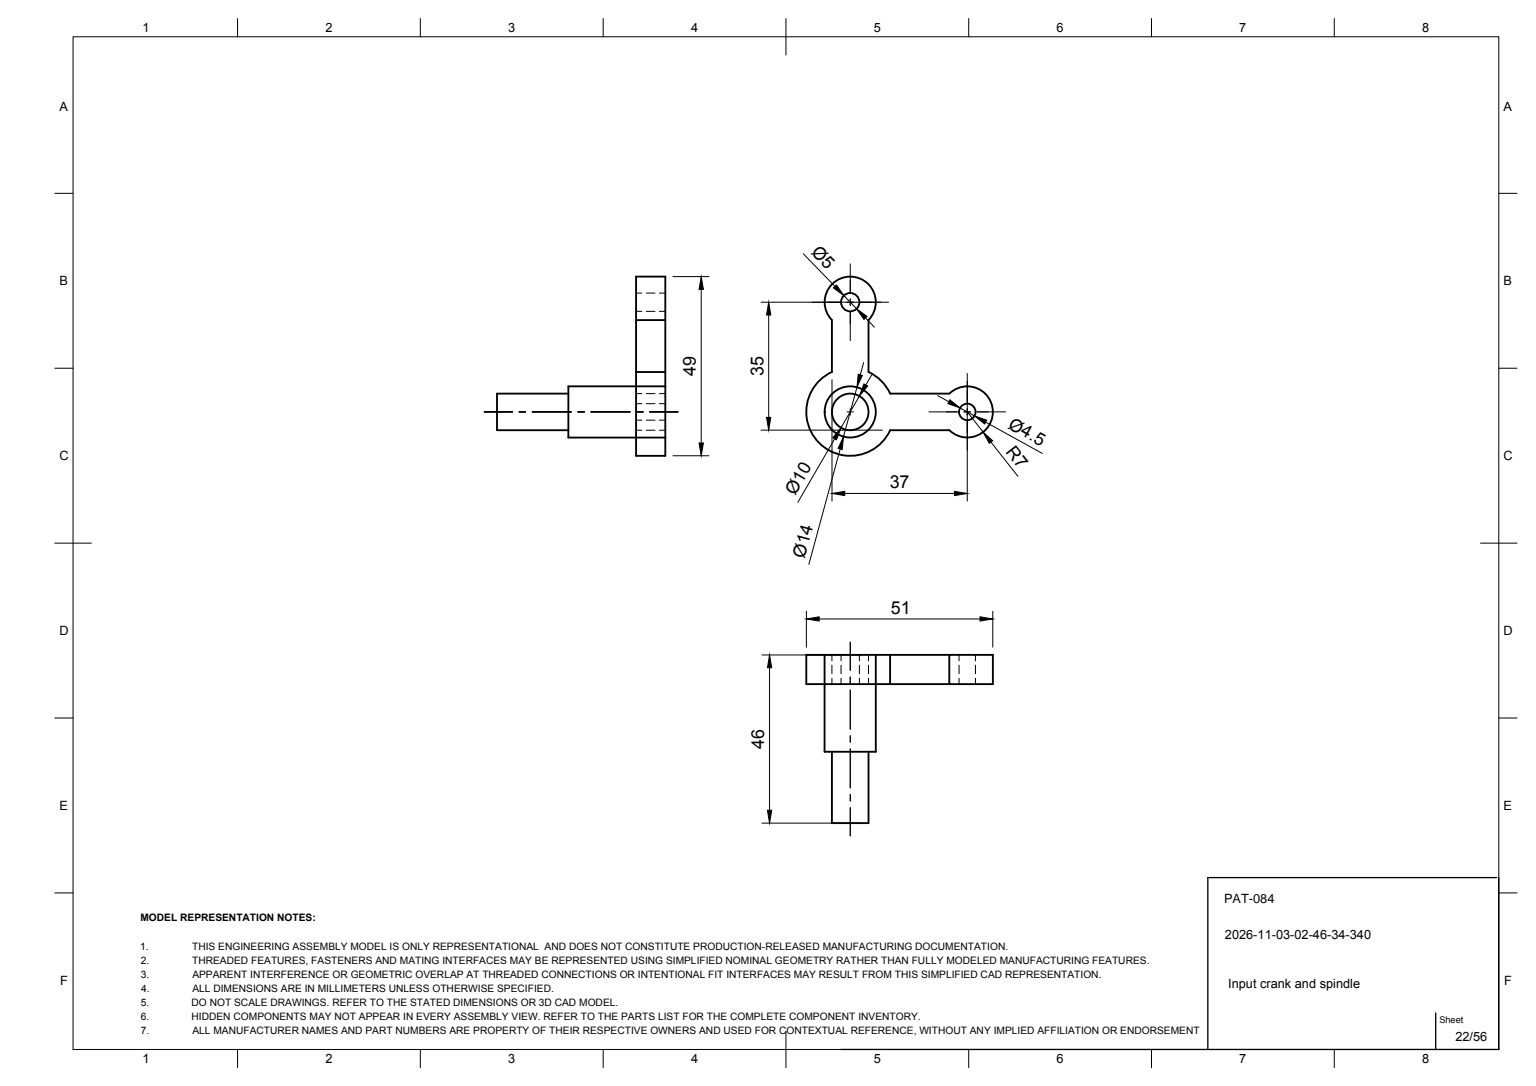
ISO-10303-21;
HEADER;
/* Generated by software containing ST-Developer
 * from STEP Tools, Inc. (www.steptools.com) 
 */

FILE_DESCRIPTION(
/* description */ ('Quick-return (Whitworth) mechanism'),
/* implementation_level */ '2;1');

FILE_NAME(
/* name */ 'Input crank and spindle.step',
/* time_stamp */ '2026-10-28T03:25:57-07:00',
/* author */ (''),
/* organization */ (''),
/* preprocessor_version */ 'ST-DEVELOPER v20.2',
/* originating_system */ 'Autodesk Translation Framework v15.17.0.0',
/* authorisation */ '');

FILE_SCHEMA (('AUTOMOTIVE_DESIGN { 1 0 10303 214 3 1 1 }'));
ENDSEC;

DATA;
#10=MECHANICAL_DESIGN_GEOMETRIC_PRESENTATION_REPRESENTATION('',(#511),#14878);
#415=SHAPE_REPRESENTATION_RELATIONSHIP('SRR','None',#15085,#459);
#459=ADVANCED_BREP_SHAPE_REPRESENTATION('',(#563),#14842);
#511=STYLED_ITEM('',(#15399),#563);
#563=MANIFOLD_SOLID_BREP('Body1',#7865);
#702=FACE_BOUND('',#1829,.T.);
#703=FACE_BOUND('',#1830,.T.);
#704=FACE_BOUND('',#1831,.T.);
#705=FACE_BOUND('',#1838,.T.);
#706=FACE_BOUND('',#1839,.T.);
#707=FACE_BOUND('',#1843,.T.);
#873=PLANE('',#8850);
#874=PLANE('',#8851);
#875=PLANE('',#8857);
#876=PLANE('',#8864);
#877=PLANE('',#8865);
#878=PLANE('',#8867);
#879=PLANE('',#8869);
#880=PLANE('',#8875);
#1248=FACE_OUTER_BOUND('',#1825,.T.);
#1249=FACE_OUTER_BOUND('',#1826,.T.);
#1250=FACE_OUTER_BOUND('',#1827,.T.);
#1251=FACE_OUTER_BOUND('',#1828,.T.);
#1252=FACE_OUTER_BOUND('',#1832,.T.);
#1253=FACE_OUTER_BOUND('',#1833,.T.);
#1254=FACE_OUTER_BOUND('',#1834,.T.);
#1255=FACE_OUTER_BOUND('',#1835,.T.);
#1256=FACE_OUTER_BOUND('',#1836,.T.);
#1257=FACE_OUTER_BOUND('',#1837,.T.);
#1258=FACE_OUTER_BOUND('',#1840,.T.);
#1259=FACE_OUTER_BOUND('',#1841,.T.);
#1260=FACE_OUTER_BOUND('',#1842,.T.);
#1261=FACE_OUTER_BOUND('',#1844,.T.);
#1262=FACE_OUTER_BOUND('',#1845,.T.);
#1263=FACE_OUTER_BOUND('',#1846,.T.);
#1825=EDGE_LOOP('',(#6130,#6131,#6132,#6133));
#1826=EDGE_LOOP('',(#6134,#6135,#6136,#6137));
#1827=EDGE_LOOP('',(#6138,#6139,#6140,#6141));
#1828=EDGE_LOOP('',(#6142,#6143,#6144,#6145,#6146,#6147,#6148,#6149));
#1829=EDGE_LOOP('',(#6150));
#1830=EDGE_LOOP('',(#6151));
#1831=EDGE_LOOP('',(#6152));
#1832=EDGE_LOOP('',(#6153,#6154,#6155,#6156));
#1833=EDGE_LOOP('',(#6157,#6158,#6159,#6160));
#1834=EDGE_LOOP('',(#6161,#6162,#6163,#6164));
#1835=EDGE_LOOP('',(#6165,#6166,#6167,#6168));
#1836=EDGE_LOOP('',(#6169,#6170,#6171,#6172));
#1837=EDGE_LOOP('',(#6173,#6174,#6175,#6176,#6177,#6178,#6179,#6180));
#1838=EDGE_LOOP('',(#6181));
#1839=EDGE_LOOP('',(#6182));
#1840=EDGE_LOOP('',(#6183,#6184,#6185,#6186));
#1841=EDGE_LOOP('',(#6187,#6188,#6189,#6190));
#1842=EDGE_LOOP('',(#6191));
#1843=EDGE_LOOP('',(#6192));
#1844=EDGE_LOOP('',(#6193,#6194,#6195,#6196));
#1845=EDGE_LOOP('',(#6197,#6198,#6199,#6200));
#1846=EDGE_LOOP('',(#6201));
#2342=LINE('',#13382,#2865);
#2343=LINE('',#13387,#2866);
#2344=LINE('',#13391,#2867);
#2345=LINE('',#13395,#2868);
#2346=LINE('',#13397,#2869);
#2347=LINE('',#13398,#2870);
#2348=LINE('',#13401,#2871);
#2349=LINE('',#13405,#2872);
#2350=LINE('',#13409,#2873);
#2351=LINE('',#13417,#2874);
#2352=LINE('',#13418,#2875);
#2353=LINE('',#13422,#2876);
#2354=LINE('',#13425,#2877);
#2355=LINE('',#13429,#2878);
#2356=LINE('',#13431,#2879);
#2357=LINE('',#13435,#2880);
#2358=LINE('',#13436,#2881);
#2359=LINE('',#13439,#2882);
#2360=LINE('',#13448,#2883);
#2361=LINE('',#13451,#2884);
#2865=VECTOR('',#10493,0.225);
#2866=VECTOR('',#10498,1.);
#2867=VECTOR('',#10501,1.);
#2868=VECTOR('',#10506,1.);
#2869=VECTOR('',#10507,1.);
#2870=VECTOR('',#10508,1.);
#2871=VECTOR('',#10511,1.);
#2872=VECTOR('',#10514,1.);
#2873=VECTOR('',#10517,1.);
#2874=VECTOR('',#10526,1.);
#2875=VECTOR('',#10527,1.);
#2876=VECTOR('',#10532,1.);
#2877=VECTOR('',#10535,0.25);
#2878=VECTOR('',#10540,1.);
#2879=VECTOR('',#10541,1.);
#2880=VECTOR('',#10546,1.);
#2881=VECTOR('',#10547,1.);
#2882=VECTOR('',#10552,1.);
#2883=VECTOR('',#10565,0.7);
#2884=VECTOR('',#10568,0.5);
#3452=CIRCLE('',#8845,0.225);
#3453=CIRCLE('',#8846,0.225);
#3454=CIRCLE('',#8848,0.7);
#3455=CIRCLE('',#8849,0.7);
#3456=CIRCLE('',#8852,1.2);
#3457=CIRCLE('',#8853,0.7);
#3458=CIRCLE('',#8854,1.2);
#3459=CIRCLE('',#8855,0.25);
#3460=CIRCLE('',#8856,0.7);
#3461=CIRCLE('',#8859,1.2);
#3462=CIRCLE('',#8861,0.25);
#3463=CIRCLE('',#8863,0.7);
#3464=CIRCLE('',#8866,1.2);
#3465=CIRCLE('',#8870,0.7);
#3466=CIRCLE('',#8871,0.5);
#3467=CIRCLE('',#8874,0.5);
#3931=VERTEX_POINT('',#13379);
#3932=VERTEX_POINT('',#13381);
#3933=VERTEX_POINT('',#13385);
#3934=VERTEX_POINT('',#13386);
#3935=VERTEX_POINT('',#13388);
#3936=VERTEX_POINT('',#13390);
#3937=VERTEX_POINT('',#13394);
#3938=VERTEX_POINT('',#13396);
#3939=VERTEX_POINT('',#13400);
#3940=VERTEX_POINT('',#13402);
#3941=VERTEX_POINT('',#13404);
#3942=VERTEX_POINT('',#13406);
#3943=VERTEX_POINT('',#13408);
#3944=VERTEX_POINT('',#13411);
#3945=VERTEX_POINT('',#13413);
#3946=VERTEX_POINT('',#13416);
#3947=VERTEX_POINT('',#13420);
#3948=VERTEX_POINT('',#13424);
#3949=VERTEX_POINT('',#13428);
#3950=VERTEX_POINT('',#13430);
#3951=VERTEX_POINT('',#13434);
#3952=VERTEX_POINT('',#13443);
#3953=VERTEX_POINT('',#13445);
#3954=VERTEX_POINT('',#13450);
#4722=EDGE_CURVE('',#3931,#3931,#3452,.T.);
#4723=EDGE_CURVE('',#3931,#3932,#2342,.T.);
#4724=EDGE_CURVE('',#3932,#3932,#3453,.T.);
#4725=EDGE_CURVE('',#3933,#3934,#2343,.T.);
#4726=EDGE_CURVE('',#3935,#3933,#3454,.T.);
#4727=EDGE_CURVE('',#3936,#3935,#2344,.T.);
#4728=EDGE_CURVE('',#3936,#3934,#3455,.T.);
#4729=EDGE_CURVE('',#3937,#3934,#2345,.T.);
#4730=EDGE_CURVE('',#3938,#3937,#2346,.T.);
#4731=EDGE_CURVE('',#3933,#3938,#2347,.T.);
#4732=EDGE_CURVE('',#3936,#3939,#2348,.T.);
#4733=EDGE_CURVE('',#3940,#3939,#3456,.T.);
#4734=EDGE_CURVE('',#3940,#3941,#2349,.T.);
#4735=EDGE_CURVE('',#3942,#3941,#3457,.T.);
#4736=EDGE_CURVE('',#3942,#3943,#2350,.T.);
#4737=EDGE_CURVE('',#3937,#3943,#3458,.T.);
#4738=EDGE_CURVE('',#3944,#3944,#3459,.T.);
#4739=EDGE_CURVE('',#3945,#3945,#3460,.T.);
#4740=EDGE_CURVE('',#3946,#3935,#2351,.T.);
#4741=EDGE_CURVE('',#3939,#3946,#2352,.T.);
#4742=EDGE_CURVE('',#3947,#3946,#3461,.T.);
#4743=EDGE_CURVE('',#3947,#3940,#2353,.T.);
#4744=EDGE_CURVE('',#3944,#3948,#2354,.T.);
#4745=EDGE_CURVE('',#3948,#3948,#3462,.T.);
#4746=EDGE_CURVE('',#3942,#3949,#2355,.T.);
#4747=EDGE_CURVE('',#3950,#3941,#2356,.T.);
#4748=EDGE_CURVE('',#3949,#3950,#3463,.T.);
#4749=EDGE_CURVE('',#3951,#3949,#2357,.T.);
#4750=EDGE_CURVE('',#3943,#3951,#2358,.T.);
#4751=EDGE_CURVE('',#3938,#3951,#3464,.T.);
#4752=EDGE_CURVE('',#3950,#3947,#2359,.T.);
#4753=EDGE_CURVE('',#3952,#3952,#3465,.T.);
#4754=EDGE_CURVE('',#3953,#3953,#3466,.T.);
#4755=EDGE_CURVE('',#3945,#3952,#2360,.T.);
#4756=EDGE_CURVE('',#3953,#3954,#2361,.T.);
#4757=EDGE_CURVE('',#3954,#3954,#3467,.T.);
#6130=ORIENTED_EDGE('',*,*,#4722,.F.);
#6131=ORIENTED_EDGE('',*,*,#4723,.T.);
#6132=ORIENTED_EDGE('',*,*,#4724,.F.);
#6133=ORIENTED_EDGE('',*,*,#4723,.F.);
#6134=ORIENTED_EDGE('',*,*,#4725,.F.);
#6135=ORIENTED_EDGE('',*,*,#4726,.F.);
#6136=ORIENTED_EDGE('',*,*,#4727,.F.);
#6137=ORIENTED_EDGE('',*,*,#4728,.T.);
#6138=ORIENTED_EDGE('',*,*,#4725,.T.);
#6139=ORIENTED_EDGE('',*,*,#4729,.F.);
#6140=ORIENTED_EDGE('',*,*,#4730,.F.);
#6141=ORIENTED_EDGE('',*,*,#4731,.F.);
#6142=ORIENTED_EDGE('',*,*,#4728,.F.);
#6143=ORIENTED_EDGE('',*,*,#4732,.T.);
#6144=ORIENTED_EDGE('',*,*,#4733,.F.);
#6145=ORIENTED_EDGE('',*,*,#4734,.T.);
#6146=ORIENTED_EDGE('',*,*,#4735,.F.);
#6147=ORIENTED_EDGE('',*,*,#4736,.T.);
#6148=ORIENTED_EDGE('',*,*,#4737,.F.);
#6149=ORIENTED_EDGE('',*,*,#4729,.T.);
#6150=ORIENTED_EDGE('',*,*,#4722,.T.);
#6151=ORIENTED_EDGE('',*,*,#4738,.T.);
#6152=ORIENTED_EDGE('',*,*,#4739,.T.);
#6153=ORIENTED_EDGE('',*,*,#4727,.T.);
#6154=ORIENTED_EDGE('',*,*,#4740,.F.);
#6155=ORIENTED_EDGE('',*,*,#4741,.F.);
#6156=ORIENTED_EDGE('',*,*,#4732,.F.);
#6157=ORIENTED_EDGE('',*,*,#4741,.T.);
#6158=ORIENTED_EDGE('',*,*,#4742,.F.);
#6159=ORIENTED_EDGE('',*,*,#4743,.T.);
#6160=ORIENTED_EDGE('',*,*,#4733,.T.);
#6161=ORIENTED_EDGE('',*,*,#4738,.F.);
#6162=ORIENTED_EDGE('',*,*,#4744,.T.);
#6163=ORIENTED_EDGE('',*,*,#4745,.F.);
#6164=ORIENTED_EDGE('',*,*,#4744,.F.);
#6165=ORIENTED_EDGE('',*,*,#4746,.F.);
#6166=ORIENTED_EDGE('',*,*,#4735,.T.);
#6167=ORIENTED_EDGE('',*,*,#4747,.F.);
#6168=ORIENTED_EDGE('',*,*,#4748,.F.);
#6169=ORIENTED_EDGE('',*,*,#4746,.T.);
#6170=ORIENTED_EDGE('',*,*,#4749,.F.);
#6171=ORIENTED_EDGE('',*,*,#4750,.F.);
#6172=ORIENTED_EDGE('',*,*,#4736,.F.);
#6173=ORIENTED_EDGE('',*,*,#4731,.T.);
#6174=ORIENTED_EDGE('',*,*,#4751,.T.);
#6175=ORIENTED_EDGE('',*,*,#4749,.T.);
#6176=ORIENTED_EDGE('',*,*,#4748,.T.);
#6177=ORIENTED_EDGE('',*,*,#4752,.T.);
#6178=ORIENTED_EDGE('',*,*,#4742,.T.);
#6179=ORIENTED_EDGE('',*,*,#4740,.T.);
#6180=ORIENTED_EDGE('',*,*,#4726,.T.);
#6181=ORIENTED_EDGE('',*,*,#4724,.T.);
#6182=ORIENTED_EDGE('',*,*,#4745,.T.);
#6183=ORIENTED_EDGE('',*,*,#4747,.T.);
#6184=ORIENTED_EDGE('',*,*,#4734,.F.);
#6185=ORIENTED_EDGE('',*,*,#4743,.F.);
#6186=ORIENTED_EDGE('',*,*,#4752,.F.);
#6187=ORIENTED_EDGE('',*,*,#4730,.T.);
#6188=ORIENTED_EDGE('',*,*,#4737,.T.);
#6189=ORIENTED_EDGE('',*,*,#4750,.T.);
#6190=ORIENTED_EDGE('',*,*,#4751,.F.);
#6191=ORIENTED_EDGE('',*,*,#4753,.F.);
#6192=ORIENTED_EDGE('',*,*,#4754,.F.);
#6193=ORIENTED_EDGE('',*,*,#4739,.F.);
#6194=ORIENTED_EDGE('',*,*,#4755,.T.);
#6195=ORIENTED_EDGE('',*,*,#4753,.T.);
#6196=ORIENTED_EDGE('',*,*,#4755,.F.);
#6197=ORIENTED_EDGE('',*,*,#4754,.T.);
#6198=ORIENTED_EDGE('',*,*,#4756,.T.);
#6199=ORIENTED_EDGE('',*,*,#4757,.T.);
#6200=ORIENTED_EDGE('',*,*,#4756,.F.);
#6201=ORIENTED_EDGE('',*,*,#4757,.F.);
#7298=CYLINDRICAL_SURFACE('',#8844,0.225);
#7299=CYLINDRICAL_SURFACE('',#8847,0.7);
#7300=CYLINDRICAL_SURFACE('',#8858,1.2);
#7301=CYLINDRICAL_SURFACE('',#8860,0.25);
#7302=CYLINDRICAL_SURFACE('',#8862,0.7);
#7303=CYLINDRICAL_SURFACE('',#8868,1.2);
#7304=CYLINDRICAL_SURFACE('',#8872,0.7);
#7305=CYLINDRICAL_SURFACE('',#8873,0.5);
#7579=ADVANCED_FACE('',(#1248),#7298,.F.);
#7580=ADVANCED_FACE('',(#1249),#7299,.T.);
#7581=ADVANCED_FACE('',(#1250),#873,.T.);
#7582=ADVANCED_FACE('',(#1251,#702,#703,#704),#874,.F.);
#7583=ADVANCED_FACE('',(#1252),#875,.T.);
#7584=ADVANCED_FACE('',(#1253),#7300,.T.);
#7585=ADVANCED_FACE('',(#1254),#7301,.F.);
#7586=ADVANCED_FACE('',(#1255),#7302,.T.);
#7587=ADVANCED_FACE('',(#1256),#876,.T.);
#7588=ADVANCED_FACE('',(#1257,#705,#706),#877,.T.);
#7589=ADVANCED_FACE('',(#1258),#878,.T.);
#7590=ADVANCED_FACE('',(#1259),#7303,.T.);
#7591=ADVANCED_FACE('',(#1260,#707),#879,.F.);
#7592=ADVANCED_FACE('',(#1261),#7304,.T.);
#7593=ADVANCED_FACE('',(#1262),#7305,.T.);
#7594=ADVANCED_FACE('',(#1263),#880,.F.);
#7865=CLOSED_SHELL('',(#7579,#7580,#7581,#7582,#7583,#7584,#7585,#7586,
#7587,#7588,#7589,#7590,#7591,#7592,#7593,#7594));
#8843=AXIS2_PLACEMENT_3D('',#13377,#10487,#10488);
#8844=AXIS2_PLACEMENT_3D('',#13378,#10489,#10490);
#8845=AXIS2_PLACEMENT_3D('',#13380,#10491,#10492);
#8846=AXIS2_PLACEMENT_3D('',#13383,#10494,#10495);
#8847=AXIS2_PLACEMENT_3D('',#13384,#10496,#10497);
#8848=AXIS2_PLACEMENT_3D('',#13389,#10499,#10500);
#8849=AXIS2_PLACEMENT_3D('',#13392,#10502,#10503);
#8850=AXIS2_PLACEMENT_3D('',#13393,#10504,#10505);
#8851=AXIS2_PLACEMENT_3D('',#13399,#10509,#10510);
#8852=AXIS2_PLACEMENT_3D('',#13403,#10512,#10513);
#8853=AXIS2_PLACEMENT_3D('',#13407,#10515,#10516);
#8854=AXIS2_PLACEMENT_3D('',#13410,#10518,#10519);
#8855=AXIS2_PLACEMENT_3D('',#13412,#10520,#10521);
#8856=AXIS2_PLACEMENT_3D('',#13414,#10522,#10523);
#8857=AXIS2_PLACEMENT_3D('',#13415,#10524,#10525);
#8858=AXIS2_PLACEMENT_3D('',#13419,#10528,#10529);
#8859=AXIS2_PLACEMENT_3D('',#13421,#10530,#10531);
#8860=AXIS2_PLACEMENT_3D('',#13423,#10533,#10534);
#8861=AXIS2_PLACEMENT_3D('',#13426,#10536,#10537);
#8862=AXIS2_PLACEMENT_3D('',#13427,#10538,#10539);
#8863=AXIS2_PLACEMENT_3D('',#13432,#10542,#10543);
#8864=AXIS2_PLACEMENT_3D('',#13433,#10544,#10545);
#8865=AXIS2_PLACEMENT_3D('',#13437,#10548,#10549);
#8866=AXIS2_PLACEMENT_3D('',#13438,#10550,#10551);
#8867=AXIS2_PLACEMENT_3D('',#13440,#10553,#10554);
#8868=AXIS2_PLACEMENT_3D('',#13441,#10555,#10556);
#8869=AXIS2_PLACEMENT_3D('',#13442,#10557,#10558);
#8870=AXIS2_PLACEMENT_3D('',#13444,#10559,#10560);
#8871=AXIS2_PLACEMENT_3D('',#13446,#10561,#10562);
#8872=AXIS2_PLACEMENT_3D('',#13447,#10563,#10564);
#8873=AXIS2_PLACEMENT_3D('',#13449,#10566,#10567);
#8874=AXIS2_PLACEMENT_3D('',#13452,#10569,#10570);
#8875=AXIS2_PLACEMENT_3D('',#13453,#10571,#10572);
#10487=DIRECTION('axis',(0.,0.,1.));
#10488=DIRECTION('refdir',(1.,0.,0.));
#10489=DIRECTION('center_axis',(0.,0.,1.));
#10490=DIRECTION('ref_axis',(1.,0.,0.));
#10491=DIRECTION('center_axis',(0.,0.,1.));
#10492=DIRECTION('ref_axis',(1.,0.,0.));
#10493=DIRECTION('',(0.,0.,1.));
#10494=DIRECTION('center_axis',(0.,0.,-1.));
#10495=DIRECTION('ref_axis',(1.,0.,0.));
#10496=DIRECTION('center_axis',(0.,0.,1.));
#10497=DIRECTION('ref_axis',(-1.,-1.22464679914735E-16,0.));
#10498=DIRECTION('',(0.,0.,-1.));
#10499=DIRECTION('center_axis',(0.,0.,1.));
#10500=DIRECTION('ref_axis',(1.,0.,0.));
#10501=DIRECTION('',(0.,0.,1.));
#10502=DIRECTION('center_axis',(0.,0.,1.));
#10503=DIRECTION('ref_axis',(1.,0.,0.));
#10504=DIRECTION('center_axis',(0.,-1.,0.));
#10505=DIRECTION('ref_axis',(1.,0.,0.));
#10506=DIRECTION('',(-1.,0.,0.));
#10507=DIRECTION('',(0.,0.,-1.));
#10508=DIRECTION('',(1.,0.,0.));
#10509=DIRECTION('center_axis',(0.,0.,1.));
#10510=DIRECTION('ref_axis',(1.,0.,0.));
#10511=DIRECTION('',(1.,0.,0.));
#10512=DIRECTION('center_axis',(0.,0.,1.));
#10513=DIRECTION('ref_axis',(1.,0.,0.));
#10514=DIRECTION('',(0.,1.,0.));
#10515=DIRECTION('center_axis',(0.,0.,1.));
#10516=DIRECTION('ref_axis',(1.,0.,0.));
#10517=DIRECTION('',(0.,-1.,0.));
#10518=DIRECTION('center_axis',(0.,0.,1.));
#10519=DIRECTION('ref_axis',(1.,0.,0.));
#10520=DIRECTION('center_axis',(0.,0.,1.));
#10521=DIRECTION('ref_axis',(1.,0.,0.));
#10522=DIRECTION('center_axis',(0.,0.,1.));
#10523=DIRECTION('ref_axis',(1.,0.,0.));
#10524=DIRECTION('center_axis',(0.,1.,0.));
#10525=DIRECTION('ref_axis',(-1.,0.,0.));
#10526=DIRECTION('',(-1.,0.,0.));
#10527=DIRECTION('',(0.,0.,1.));
#10528=DIRECTION('center_axis',(0.,0.,1.));
#10529=DIRECTION('ref_axis',(1.,0.,0.));
#10530=DIRECTION('center_axis',(0.,0.,1.));
#10531=DIRECTION('ref_axis',(1.,0.,0.));
#10532=DIRECTION('',(0.,0.,-1.));
#10533=DIRECTION('center_axis',(0.,0.,1.));
#10534=DIRECTION('ref_axis',(1.,0.,0.));
#10535=DIRECTION('',(0.,0.,1.));
#10536=DIRECTION('center_axis',(0.,0.,-1.));
#10537=DIRECTION('ref_axis',(1.,0.,0.));
#10538=DIRECTION('center_axis',(0.,0.,1.));
#10539=DIRECTION('ref_axis',(6.12323399573677E-17,1.,0.));
#10540=DIRECTION('',(0.,0.,1.));
#10541=DIRECTION('',(0.,0.,-1.));
#10542=DIRECTION('center_axis',(0.,0.,1.));
#10543=DIRECTION('ref_axis',(1.,0.,0.));
#10544=DIRECTION('center_axis',(1.,0.,0.));
#10545=DIRECTION('ref_axis',(0.,1.,0.));
#10546=DIRECTION('',(0.,1.,0.));
#10547=DIRECTION('',(0.,0.,1.));
#10548=DIRECTION('center_axis',(0.,0.,1.));
#10549=DIRECTION('ref_axis',(1.,0.,0.));
#10550=DIRECTION('center_axis',(0.,0.,1.));
#10551=DIRECTION('ref_axis',(1.,0.,0.));
#10552=DIRECTION('',(0.,-1.,0.));
#10553=DIRECTION('center_axis',(-1.,0.,0.));
#10554=DIRECTION('ref_axis',(0.,-1.,0.));
#10555=DIRECTION('center_axis',(0.,0.,1.));
#10556=DIRECTION('ref_axis',(1.,0.,0.));
#10557=DIRECTION('center_axis',(0.,0.,1.));
#10558=DIRECTION('ref_axis',(1.,0.,0.));
#10559=DIRECTION('center_axis',(0.,0.,1.));
#10560=DIRECTION('ref_axis',(1.,0.,0.));
#10561=DIRECTION('center_axis',(0.,0.,-1.));
#10562=DIRECTION('ref_axis',(1.,0.,0.));
#10563=DIRECTION('center_axis',(0.,0.,1.));
#10564=DIRECTION('ref_axis',(1.,0.,0.));
#10565=DIRECTION('',(0.,0.,-1.));
#10566=DIRECTION('center_axis',(0.,0.,1.));
#10567=DIRECTION('ref_axis',(1.,0.,0.));
#10568=DIRECTION('',(0.,0.,-1.));
#10569=DIRECTION('center_axis',(0.,0.,1.));
#10570=DIRECTION('ref_axis',(1.,0.,0.));
#10571=DIRECTION('center_axis',(0.,0.,1.));
#10572=DIRECTION('ref_axis',(1.,0.,0.));
#13377=CARTESIAN_POINT('',(0.,0.,0.));
#13378=CARTESIAN_POINT('Origin',(-3.2,6.,4.7));
#13379=CARTESIAN_POINT('',(-3.425,6.,4.8));
#13380=CARTESIAN_POINT('Origin',(-3.2,6.,4.8));
#13381=CARTESIAN_POINT('',(-3.425,6.,5.6));
#13382=CARTESIAN_POINT('',(-3.425,6.,4.7));
#13383=CARTESIAN_POINT('Origin',(-3.2,6.,5.6));
#13384=CARTESIAN_POINT('Origin',(-3.2,6.,4.8));
#13385=CARTESIAN_POINT('',(-2.71010205144336,5.5,5.6));
#13386=CARTESIAN_POINT('',(-2.71010205144336,5.5,4.8));
#13387=CARTESIAN_POINT('',(-2.71010205144336,5.5,4.8));
#13388=CARTESIAN_POINT('',(-2.71010205144336,6.5,5.6));
#13389=CARTESIAN_POINT('Origin',(-3.2,6.,5.6));
#13390=CARTESIAN_POINT('',(-2.71010205144336,6.5,4.8));
#13391=CARTESIAN_POINT('',(-2.71010205144336,6.5,4.8));
#13392=CARTESIAN_POINT('Origin',(-3.2,6.,4.8));
#13393=CARTESIAN_POINT('Origin',(-3.2,5.5,4.8));
#13394=CARTESIAN_POINT('',(-1.09087121146357,5.5,4.8));
#13395=CARTESIAN_POINT('',(0.,5.5,4.8));
#13396=CARTESIAN_POINT('',(-1.09087121146357,5.5,5.6));
#13397=CARTESIAN_POINT('',(-1.09087121146357,5.5,4.8));
#13398=CARTESIAN_POINT('',(0.,5.5,5.6));
#13399=CARTESIAN_POINT('Origin',(0.,6.,4.8));
#13400=CARTESIAN_POINT('',(-1.09087121146357,6.5,4.8));
#13401=CARTESIAN_POINT('',(-3.2,6.5,4.8));
#13402=CARTESIAN_POINT('',(-0.5,7.09087121146357,4.8));
#13403=CARTESIAN_POINT('Origin',(0.,6.,4.8));
#13404=CARTESIAN_POINT('',(-0.5,8.51010205144336,4.8));
#13405=CARTESIAN_POINT('',(-0.5,6.,4.8));
#13406=CARTESIAN_POINT('',(0.5,8.51010205144336,4.8));
#13407=CARTESIAN_POINT('Origin',(0.,9.,4.8));
#13408=CARTESIAN_POINT('',(0.5,7.09087121146357,4.8));
#13409=CARTESIAN_POINT('',(0.5,9.,4.8));
#13410=CARTESIAN_POINT('Origin',(0.,6.,4.8));
#13411=CARTESIAN_POINT('',(-0.25,9.,4.8));
#13412=CARTESIAN_POINT('Origin',(0.,9.,4.8));
#13413=CARTESIAN_POINT('',(-0.7,6.,4.8));
#13414=CARTESIAN_POINT('Origin',(0.,6.,4.8));
#13415=CARTESIAN_POINT('Origin',(0.,6.5,4.8));
#13416=CARTESIAN_POINT('',(-1.09087121146357,6.5,5.6));
#13417=CARTESIAN_POINT('',(-3.2,6.5,5.6));
#13418=CARTESIAN_POINT('',(-1.09087121146357,6.5,4.8));
#13419=CARTESIAN_POINT('Origin',(0.,6.,4.8));
#13420=CARTESIAN_POINT('',(-0.5,7.09087121146357,5.6));
#13421=CARTESIAN_POINT('Origin',(0.,6.,5.6));
#13422=CARTESIAN_POINT('',(-0.5,7.09087121146357,4.8));
#13423=CARTESIAN_POINT('Origin',(0.,9.,4.7));
#13424=CARTESIAN_POINT('',(-0.25,9.,5.6));
#13425=CARTESIAN_POINT('',(-0.25,9.,4.7));
#13426=CARTESIAN_POINT('Origin',(0.,9.,5.6));
#13427=CARTESIAN_POINT('Origin',(0.,9.,4.8));
#13428=CARTESIAN_POINT('',(0.5,8.51010205144336,5.6));
#13429=CARTESIAN_POINT('',(0.5,8.51010205144336,4.8));
#13430=CARTESIAN_POINT('',(-0.5,8.51010205144336,5.6));
#13431=CARTESIAN_POINT('',(-0.5,8.51010205144336,4.8));
#13432=CARTESIAN_POINT('Origin',(0.,9.,5.6));
#13433=CARTESIAN_POINT('Origin',(0.5,6.,4.8));
#13434=CARTESIAN_POINT('',(0.5,7.09087121146357,5.6));
#13435=CARTESIAN_POINT('',(0.5,9.,5.6));
#13436=CARTESIAN_POINT('',(0.5,7.09087121146357,4.8));
#13437=CARTESIAN_POINT('Origin',(0.,6.,5.6));
#13438=CARTESIAN_POINT('Origin',(0.,6.,5.6));
#13439=CARTESIAN_POINT('',(-0.5,6.,5.6));
#13440=CARTESIAN_POINT('Origin',(-0.5,9.,4.8));
#13441=CARTESIAN_POINT('Origin',(0.,6.,4.8));
#13442=CARTESIAN_POINT('Origin',(0.,6.,2.95));
#13443=CARTESIAN_POINT('',(-0.7,6.,2.95));
#13444=CARTESIAN_POINT('Origin',(0.,6.,2.95));
#13445=CARTESIAN_POINT('',(-0.5,6.,2.95));
#13446=CARTESIAN_POINT('Origin',(0.,6.,2.95));
#13447=CARTESIAN_POINT('Origin',(0.,6.,2.95));
#13448=CARTESIAN_POINT('',(-0.7,6.,2.95));
#13449=CARTESIAN_POINT('Origin',(0.,6.,1.));
#13450=CARTESIAN_POINT('',(-0.5,6.,1.));
#13451=CARTESIAN_POINT('',(-0.5,6.,1.));
#13452=CARTESIAN_POINT('Origin',(0.,6.,1.));
#13453=CARTESIAN_POINT('Origin',(0.,6.,1.));
#14788=UNCERTAINTY_MEASURE_WITH_UNIT(LENGTH_MEASURE(0.001),#14879,
'DISTANCE_ACCURACY_VALUE',
'Maximum model space distance between geometric entities at asserted c
onnectivities');
#14824=UNCERTAINTY_MEASURE_WITH_UNIT(LENGTH_MEASURE(0.001),#14879,
'DISTANCE_ACCURACY_VALUE',
'Maximum model space distance between geometric entities at asserted c
onnectivities');
#14842=(
GEOMETRIC_REPRESENTATION_CONTEXT(3)
GLOBAL_UNCERTAINTY_ASSIGNED_CONTEXT((#14788))
GLOBAL_UNIT_ASSIGNED_CONTEXT((#14879,#14881,#14882))
REPRESENTATION_CONTEXT('','3D')
);
#14878=(
GEOMETRIC_REPRESENTATION_CONTEXT(3)
GLOBAL_UNCERTAINTY_ASSIGNED_CONTEXT((#14824))
GLOBAL_UNIT_ASSIGNED_CONTEXT((#14879,#14881,#14882))
REPRESENTATION_CONTEXT('','3D')
);
#14879=(
LENGTH_UNIT()
NAMED_UNIT(*)
SI_UNIT(.CENTI.,.METRE.)
);
#14881=(
NAMED_UNIT(*)
PLANE_ANGLE_UNIT()
SI_UNIT($,.RADIAN.)
);
#14882=(
NAMED_UNIT(*)
SI_UNIT($,.STERADIAN.)
SOLID_ANGLE_UNIT()
);
#14900=SHAPE_DEFINITION_REPRESENTATION(#14958,#15085);
#14958=PRODUCT_DEFINITION_SHAPE('',$,#15139);
#15085=SHAPE_REPRESENTATION('',(#8843),#14842);
#15121=PRODUCT_DEFINITION_CONTEXT('part definition',#15282,'design');
#15139=PRODUCT_DEFINITION('Input crank and spindle',
'Input crank and spindle',#15192,#15121);
#15192=PRODUCT_DEFINITION_FORMATION('',$,#15301);
#15282=APPLICATION_CONTEXT(
'Core Data for Automotive Mechanical Design Process');
#15283=PRODUCT_CONTEXT('part definition',#15282,'mechanical');
#15301=PRODUCT('Input crank and spindle','Input crank and spindle',
'Input crank and spindle',(#15283));
#15393=COLOUR_RGB('Sky Blue',0.24,0.69,0.87);
#15394=FILL_AREA_STYLE_COLOUR('',#15393);
#15395=FILL_AREA_STYLE('',(#15394));
#15396=SURFACE_STYLE_FILL_AREA(#15395);
#15397=SURFACE_SIDE_STYLE('',(#15396));
#15398=SURFACE_STYLE_USAGE(.BOTH.,#15397);
#15399=PRESENTATION_STYLE_ASSIGNMENT((#15398));
ENDSEC;
END-ISO-10303-21;
